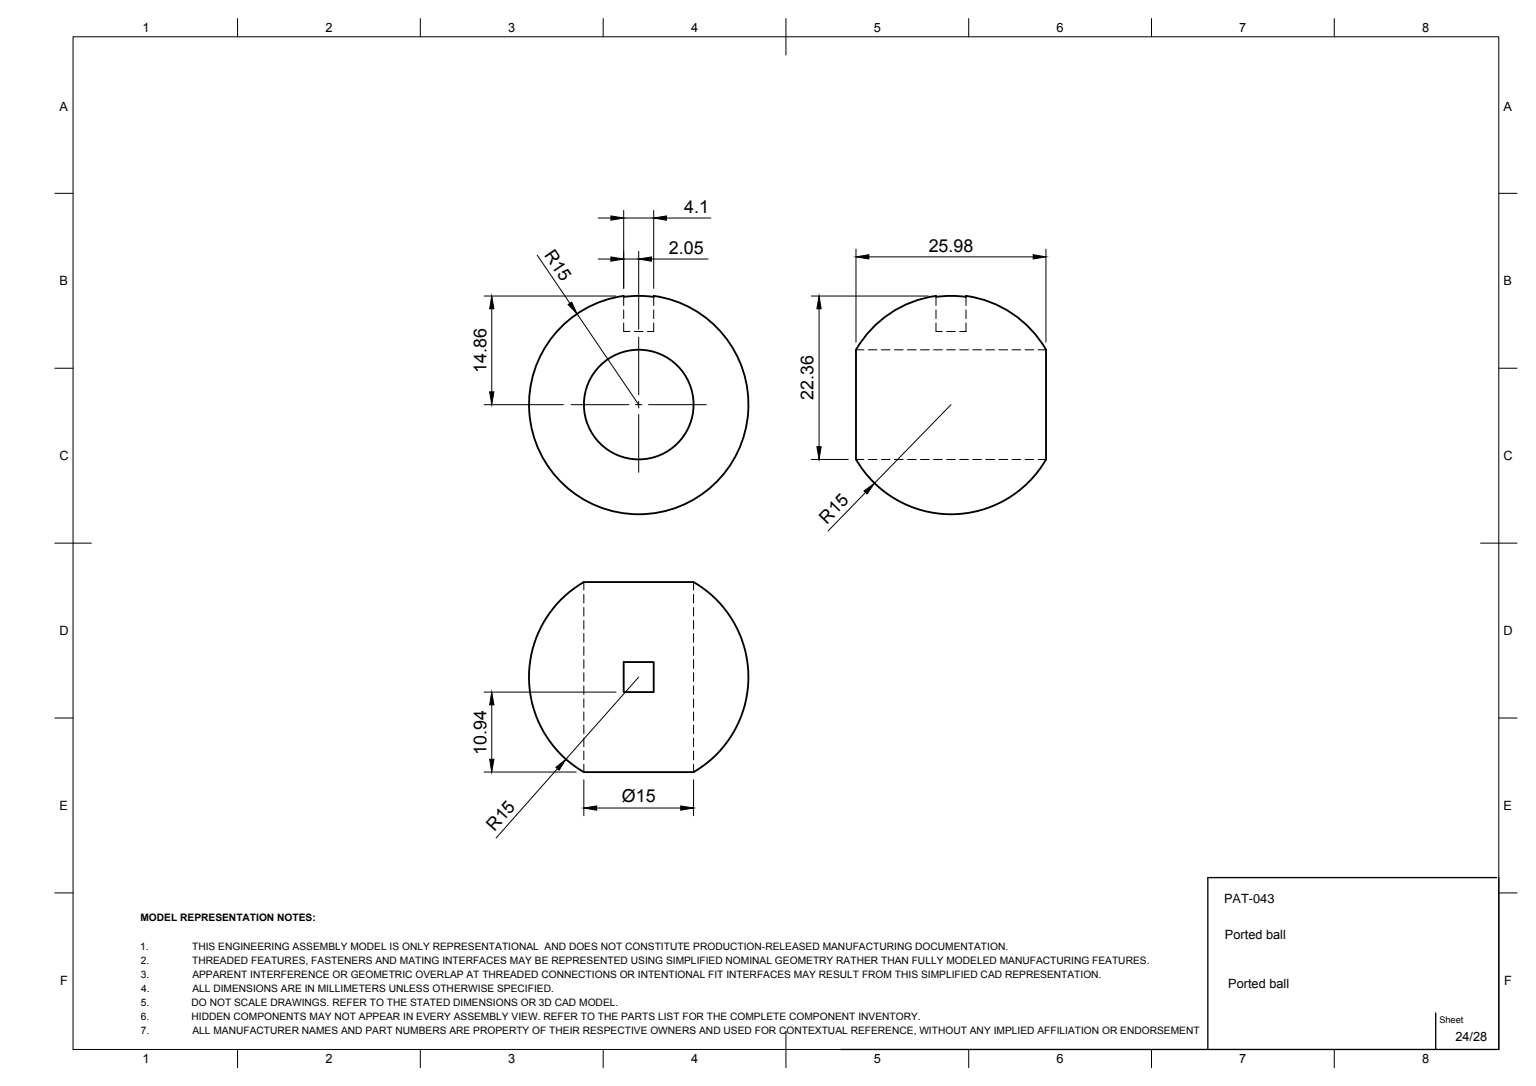
ISO-10303-21;
HEADER;
/* Generated by software containing ST-Developer
 * from STEP Tools, Inc. (www.steptools.com) 
 */

FILE_DESCRIPTION(
/* description */ ('Four-valve pipe header'),
/* implementation_level */ '2;1');

FILE_NAME(
/* name */ 'Ported ball.step',
/* time_stamp */ '2026-10-29T16:56:19-07:00',
/* author */ (''),
/* organization */ (''),
/* preprocessor_version */ 'ST-DEVELOPER v20.2',
/* originating_system */ 'Autodesk Translation Framework v15.17.0.0',
/* authorisation */ '');

FILE_SCHEMA (('AUTOMOTIVE_DESIGN { 1 0 10303 214 3 1 1 }'));
ENDSEC;

DATA;
#10=MECHANICAL_DESIGN_GEOMETRIC_PRESENTATION_REPRESENTATION('',(#353),#10119);
#245=SPHERICAL_SURFACE('',#6425,1.5);
#301=SHAPE_REPRESENTATION_RELATIONSHIP('SRR','None',#10264,#327);
#327=ADVANCED_BREP_SHAPE_REPRESENTATION('',(#377),#10113);
#353=STYLED_ITEM('',(#10456),#377);
#377=MANIFOLD_SOLID_BREP('Body1',#5601);
#526=FACE_BOUND('',#1453,.T.);
#527=FACE_BOUND('',#1454,.T.);
#693=PLANE('',#6412);
#694=PLANE('',#6414);
#695=PLANE('',#6417);
#696=PLANE('',#6419);
#697=PLANE('',#6421);
#1014=FACE_OUTER_BOUND('',#1446,.T.);
#1015=FACE_OUTER_BOUND('',#1447,.T.);
#1016=FACE_OUTER_BOUND('',#1448,.T.);
#1017=FACE_OUTER_BOUND('',#1449,.T.);
#1018=FACE_OUTER_BOUND('',#1450,.T.);
#1019=FACE_OUTER_BOUND('',#1451,.T.);
#1020=FACE_OUTER_BOUND('',#1452,.T.);
#1446=EDGE_LOOP('',(#4879,#4880,#4881,#4882));
#1447=EDGE_LOOP('',(#4883,#4884,#4885,#4886,#4887));
#1448=EDGE_LOOP('',(#4888,#4889,#4890,#4891));
#1449=EDGE_LOOP('',(#4892,#4893,#4894,#4895));
#1450=EDGE_LOOP('',(#4896,#4897,#4898,#4899));
#1451=EDGE_LOOP('',(#4900,#4901,#4902,#4903));
#1452=EDGE_LOOP('',(#4904,#4905,#4906,#4907,#4908,#4909,#4910));
#1453=EDGE_LOOP('',(#4911));
#1454=EDGE_LOOP('',(#4912));
#1834=LINE('',#9715,#2252);
#1835=LINE('',#9717,#2253);
#1836=LINE('',#9718,#2254);
#1837=LINE('',#9723,#2255);
#1838=LINE('',#9725,#2256);
#1839=LINE('',#9731,#2257);
#1840=LINE('',#9732,#2258);
#1841=LINE('',#9735,#2259);
#1842=LINE('',#9741,#2260);
#2252=VECTOR('',#7921,1.);
#2253=VECTOR('',#7922,1.);
#2254=VECTOR('',#7923,1.);
#2255=VECTOR('',#7928,1.);
#2256=VECTOR('',#7929,1.);
#2257=VECTOR('',#7936,1.);
#2258=VECTOR('',#7937,1.);
#2259=VECTOR('',#7942,1.);
#2260=VECTOR('',#7949,0.75);
#2549=CIRCLE('',#6413,1.48592563743951);
#2550=CIRCLE('',#6415,1.48592563743951);
#2551=CIRCLE('',#6416,1.48592563743951);
#2552=CIRCLE('',#6418,1.48592563743951);
#2553=CIRCLE('',#6420,1.48592563743951);
#2554=CIRCLE('',#6423,0.75);
#2555=CIRCLE('',#6424,0.75);
#2556=CIRCLE('',#6426,1.5);
#2950=VERTEX_POINT('',#9711);
#2951=VERTEX_POINT('',#9712);
#2952=VERTEX_POINT('',#9714);
#2953=VERTEX_POINT('',#9716);
#2954=VERTEX_POINT('',#9720);
#2955=VERTEX_POINT('',#9722);
#2956=VERTEX_POINT('',#9724);
#2957=VERTEX_POINT('',#9728);
#2958=VERTEX_POINT('',#9730);
#2959=VERTEX_POINT('',#9738);
#2960=VERTEX_POINT('',#9740);
#2961=VERTEX_POINT('',#9744);
#3606=EDGE_CURVE('',#2950,#2951,#2549,.T.);
#3607=EDGE_CURVE('',#2952,#2950,#1834,.T.);
#3608=EDGE_CURVE('',#2953,#2952,#1835,.T.);
#3609=EDGE_CURVE('',#2953,#2951,#1836,.T.);
#3610=EDGE_CURVE('',#2951,#2954,#2550,.T.);
#3611=EDGE_CURVE('',#2955,#2953,#1837,.T.);
#3612=EDGE_CURVE('',#2955,#2956,#1838,.T.);
#3613=EDGE_CURVE('',#2954,#2956,#2551,.T.);
#3614=EDGE_CURVE('',#2956,#2957,#2552,.T.);
#3615=EDGE_CURVE('',#2958,#2955,#1839,.T.);
#3616=EDGE_CURVE('',#2958,#2957,#1840,.T.);
#3617=EDGE_CURVE('',#2957,#2950,#2553,.T.);
#3618=EDGE_CURVE('',#2952,#2958,#1841,.T.);
#3619=EDGE_CURVE('',#2959,#2959,#2554,.T.);
#3620=EDGE_CURVE('',#2959,#2960,#1842,.T.);
#3621=EDGE_CURVE('',#2960,#2960,#2555,.T.);
#3622=EDGE_CURVE('',#2954,#2961,#2556,.T.);
#4879=ORIENTED_EDGE('',*,*,#3606,.F.);
#4880=ORIENTED_EDGE('',*,*,#3607,.F.);
#4881=ORIENTED_EDGE('',*,*,#3608,.F.);
#4882=ORIENTED_EDGE('',*,*,#3609,.T.);
#4883=ORIENTED_EDGE('',*,*,#3610,.F.);
#4884=ORIENTED_EDGE('',*,*,#3609,.F.);
#4885=ORIENTED_EDGE('',*,*,#3611,.F.);
#4886=ORIENTED_EDGE('',*,*,#3612,.T.);
#4887=ORIENTED_EDGE('',*,*,#3613,.F.);
#4888=ORIENTED_EDGE('',*,*,#3614,.F.);
#4889=ORIENTED_EDGE('',*,*,#3612,.F.);
#4890=ORIENTED_EDGE('',*,*,#3615,.F.);
#4891=ORIENTED_EDGE('',*,*,#3616,.T.);
#4892=ORIENTED_EDGE('',*,*,#3617,.F.);
#4893=ORIENTED_EDGE('',*,*,#3616,.F.);
#4894=ORIENTED_EDGE('',*,*,#3618,.F.);
#4895=ORIENTED_EDGE('',*,*,#3607,.T.);
#4896=ORIENTED_EDGE('',*,*,#3611,.T.);
#4897=ORIENTED_EDGE('',*,*,#3608,.T.);
#4898=ORIENTED_EDGE('',*,*,#3618,.T.);
#4899=ORIENTED_EDGE('',*,*,#3615,.T.);
#4900=ORIENTED_EDGE('',*,*,#3619,.F.);
#4901=ORIENTED_EDGE('',*,*,#3620,.T.);
#4902=ORIENTED_EDGE('',*,*,#3621,.F.);
#4903=ORIENTED_EDGE('',*,*,#3620,.F.);
#4904=ORIENTED_EDGE('',*,*,#3614,.T.);
#4905=ORIENTED_EDGE('',*,*,#3617,.T.);
#4906=ORIENTED_EDGE('',*,*,#3606,.T.);
#4907=ORIENTED_EDGE('',*,*,#3610,.T.);
#4908=ORIENTED_EDGE('',*,*,#3622,.T.);
#4909=ORIENTED_EDGE('',*,*,#3622,.F.);
#4910=ORIENTED_EDGE('',*,*,#3613,.T.);
#4911=ORIENTED_EDGE('',*,*,#3621,.T.);
#4912=ORIENTED_EDGE('',*,*,#3619,.T.);
#5240=CYLINDRICAL_SURFACE('',#6422,0.75);
#5514=ADVANCED_FACE('',(#1014),#693,.F.);
#5515=ADVANCED_FACE('',(#1015),#694,.F.);
#5516=ADVANCED_FACE('',(#1016),#695,.F.);
#5517=ADVANCED_FACE('',(#1017),#696,.F.);
#5518=ADVANCED_FACE('',(#1018),#697,.T.);
#5519=ADVANCED_FACE('',(#1019),#5240,.F.);
#5520=ADVANCED_FACE('',(#1020,#526,#527),#245,.T.);
#5601=CLOSED_SHELL('',(#5514,#5515,#5516,#5517,#5518,#5519,#5520));
#6411=AXIS2_PLACEMENT_3D('',#9709,#7915,#7916);
#6412=AXIS2_PLACEMENT_3D('',#9710,#7917,#7918);
#6413=AXIS2_PLACEMENT_3D('',#9713,#7919,#7920);
#6414=AXIS2_PLACEMENT_3D('',#9719,#7924,#7925);
#6415=AXIS2_PLACEMENT_3D('',#9721,#7926,#7927);
#6416=AXIS2_PLACEMENT_3D('',#9726,#7930,#7931);
#6417=AXIS2_PLACEMENT_3D('',#9727,#7932,#7933);
#6418=AXIS2_PLACEMENT_3D('',#9729,#7934,#7935);
#6419=AXIS2_PLACEMENT_3D('',#9733,#7938,#7939);
#6420=AXIS2_PLACEMENT_3D('',#9734,#7940,#7941);
#6421=AXIS2_PLACEMENT_3D('',#9736,#7943,#7944);
#6422=AXIS2_PLACEMENT_3D('',#9737,#7945,#7946);
#6423=AXIS2_PLACEMENT_3D('',#9739,#7947,#7948);
#6424=AXIS2_PLACEMENT_3D('',#9742,#7950,#7951);
#6425=AXIS2_PLACEMENT_3D('',#9743,#7952,#7953);
#6426=AXIS2_PLACEMENT_3D('',#9745,#7954,#7955);
#7915=DIRECTION('axis',(0.,0.,1.));
#7916=DIRECTION('refdir',(1.,0.,0.));
#7917=DIRECTION('center_axis',(0.,-1.,0.));
#7918=DIRECTION('ref_axis',(1.,0.,0.));
#7919=DIRECTION('center_axis',(0.,-1.,0.));
#7920=DIRECTION('ref_axis',(0.,0.,1.));
#7921=DIRECTION('',(0.,0.,1.));
#7922=DIRECTION('',(1.,0.,0.));
#7923=DIRECTION('',(0.,0.,1.));
#7924=DIRECTION('center_axis',(-1.,0.,0.));
#7925=DIRECTION('ref_axis',(0.,-1.,0.));
#7926=DIRECTION('center_axis',(-1.,0.,0.));
#7927=DIRECTION('ref_axis',(0.,0.,-1.));
#7928=DIRECTION('',(0.,-1.,0.));
#7929=DIRECTION('',(0.,0.,1.));
#7930=DIRECTION('center_axis',(-1.,0.,0.));
#7931=DIRECTION('ref_axis',(0.,0.,-1.));
#7932=DIRECTION('center_axis',(0.,1.,0.));
#7933=DIRECTION('ref_axis',(-1.,0.,0.));
#7934=DIRECTION('center_axis',(0.,1.,0.));
#7935=DIRECTION('ref_axis',(0.,0.,-1.));
#7936=DIRECTION('',(-1.,0.,0.));
#7937=DIRECTION('',(0.,0.,1.));
#7938=DIRECTION('center_axis',(1.,0.,0.));
#7939=DIRECTION('ref_axis',(0.,1.,0.));
#7940=DIRECTION('center_axis',(1.,0.,0.));
#7941=DIRECTION('ref_axis',(0.,0.,1.));
#7942=DIRECTION('',(0.,1.,0.));
#7943=DIRECTION('center_axis',(0.,0.,1.));
#7944=DIRECTION('ref_axis',(1.,0.,0.));
#7945=DIRECTION('center_axis',(0.,1.,0.));
#7946=DIRECTION('ref_axis',(1.,0.,0.));
#7947=DIRECTION('center_axis',(0.,1.,0.));
#7948=DIRECTION('ref_axis',(1.,0.,0.));
#7949=DIRECTION('',(0.,1.,0.));
#7950=DIRECTION('center_axis',(0.,-1.,0.));
#7951=DIRECTION('ref_axis',(1.,0.,0.));
#7952=DIRECTION('center_axis',(6.12323399573677E-17,0.,1.));
#7953=DIRECTION('ref_axis',(1.,0.,0.));
#7954=DIRECTION('center_axis',(1.22464679914735E-16,-1.,0.));
#7955=DIRECTION('ref_axis',(-1.,-1.22464679914735E-16,0.));
#9709=CARTESIAN_POINT('',(0.,0.,0.));
#9710=CARTESIAN_POINT('Origin',(-0.205,-0.205,6.));
#9711=CARTESIAN_POINT('',(0.205,-0.205,6.47171668469172));
#9712=CARTESIAN_POINT('',(-0.205,-0.205,6.47171668469172));
#9713=CARTESIAN_POINT('Origin',(0.,-0.205,5.));
#9714=CARTESIAN_POINT('',(0.205,-0.205,6.));
#9715=CARTESIAN_POINT('',(0.205,-0.205,6.));
#9716=CARTESIAN_POINT('',(-0.205,-0.205,6.));
#9717=CARTESIAN_POINT('',(-0.205,-0.205,6.));
#9718=CARTESIAN_POINT('',(-0.205,-0.205,6.));
#9719=CARTESIAN_POINT('Origin',(-0.205,0.205,6.));
#9720=CARTESIAN_POINT('',(-0.205,-2.51052593825207E-17,6.48592563743951));
#9721=CARTESIAN_POINT('Origin',(-0.205,0.,5.));
#9722=CARTESIAN_POINT('',(-0.205,0.205,6.));
#9723=CARTESIAN_POINT('',(-0.205,0.205,6.));
#9724=CARTESIAN_POINT('',(-0.205,0.205,6.47171668469172));
#9725=CARTESIAN_POINT('',(-0.205,0.205,6.));
#9726=CARTESIAN_POINT('Origin',(-0.205,0.,5.));
#9727=CARTESIAN_POINT('Origin',(0.205,0.205,6.));
#9728=CARTESIAN_POINT('',(0.205,0.205,6.47171668469172));
#9729=CARTESIAN_POINT('Origin',(0.,0.205,5.));
#9730=CARTESIAN_POINT('',(0.205,0.205,6.));
#9731=CARTESIAN_POINT('',(0.205,0.205,6.));
#9732=CARTESIAN_POINT('',(0.205,0.205,6.));
#9733=CARTESIAN_POINT('Origin',(0.205,-0.205,6.));
#9734=CARTESIAN_POINT('Origin',(0.205,0.,5.));
#9735=CARTESIAN_POINT('',(0.205,-0.205,6.));
#9736=CARTESIAN_POINT('Origin',(0.,0.,6.));
#9737=CARTESIAN_POINT('Origin',(0.,-1.6,5.));
#9738=CARTESIAN_POINT('',(-0.75,-1.29903810567666,5.));
#9739=CARTESIAN_POINT('Origin',(0.,-1.29903810567666,5.));
#9740=CARTESIAN_POINT('',(-0.75,1.29903810567666,5.));
#9741=CARTESIAN_POINT('',(-0.75,-1.6,5.));
#9742=CARTESIAN_POINT('Origin',(0.,1.29903810567666,5.));
#9743=CARTESIAN_POINT('Origin',(0.,0.,5.));
#9744=CARTESIAN_POINT('',(-9.18485099360515E-17,-1.12481983699639E-32,3.5));
#9745=CARTESIAN_POINT('Origin',(0.,0.,5.));
#10082=UNCERTAINTY_MEASURE_WITH_UNIT(LENGTH_MEASURE(0.001),#10120,
'DISTANCE_ACCURACY_VALUE',
'Maximum model space distance between geometric entities at asserted c
onnectivities');
#10088=UNCERTAINTY_MEASURE_WITH_UNIT(LENGTH_MEASURE(0.001),#10120,
'DISTANCE_ACCURACY_VALUE',
'Maximum model space distance between geometric entities at asserted c
onnectivities');
#10113=(
GEOMETRIC_REPRESENTATION_CONTEXT(3)
GLOBAL_UNCERTAINTY_ASSIGNED_CONTEXT((#10082))
GLOBAL_UNIT_ASSIGNED_CONTEXT((#10120,#10122,#10123))
REPRESENTATION_CONTEXT('','3D')
);
#10119=(
GEOMETRIC_REPRESENTATION_CONTEXT(3)
GLOBAL_UNCERTAINTY_ASSIGNED_CONTEXT((#10088))
GLOBAL_UNIT_ASSIGNED_CONTEXT((#10120,#10122,#10123))
REPRESENTATION_CONTEXT('','3D')
);
#10120=(
LENGTH_UNIT()
NAMED_UNIT(*)
SI_UNIT(.CENTI.,.METRE.)
);
#10122=(
NAMED_UNIT(*)
PLANE_ANGLE_UNIT()
SI_UNIT($,.RADIAN.)
);
#10123=(
NAMED_UNIT(*)
SI_UNIT($,.STERADIAN.)
SOLID_ANGLE_UNIT()
);
#10148=SHAPE_DEFINITION_REPRESENTATION(#10178,#10264);
#10178=PRODUCT_DEFINITION_SHAPE('',$,#10295);
#10264=SHAPE_REPRESENTATION('',(#6411),#10113);
#10270=PRODUCT_DEFINITION_CONTEXT('part definition',#10362,'design');
#10295=PRODUCT_DEFINITION('Ported ball','Ported ball',#10325,#10270);
#10325=PRODUCT_DEFINITION_FORMATION('',$,#10388);
#10362=APPLICATION_CONTEXT(
'Core Data for Automotive Mechanical Design Process');
#10363=PRODUCT_CONTEXT('part definition',#10362,'mechanical');
#10388=PRODUCT('Ported ball','Ported ball','Ported ball',(#10363));
#10450=COLOUR_RGB('Light Blue',0.38,0.62,0.78);
#10451=FILL_AREA_STYLE_COLOUR('',#10450);
#10452=FILL_AREA_STYLE('',(#10451));
#10453=SURFACE_STYLE_FILL_AREA(#10452);
#10454=SURFACE_SIDE_STYLE('',(#10453));
#10455=SURFACE_STYLE_USAGE(.BOTH.,#10454);
#10456=PRESENTATION_STYLE_ASSIGNMENT((#10455));
ENDSEC;
END-ISO-10303-21;
